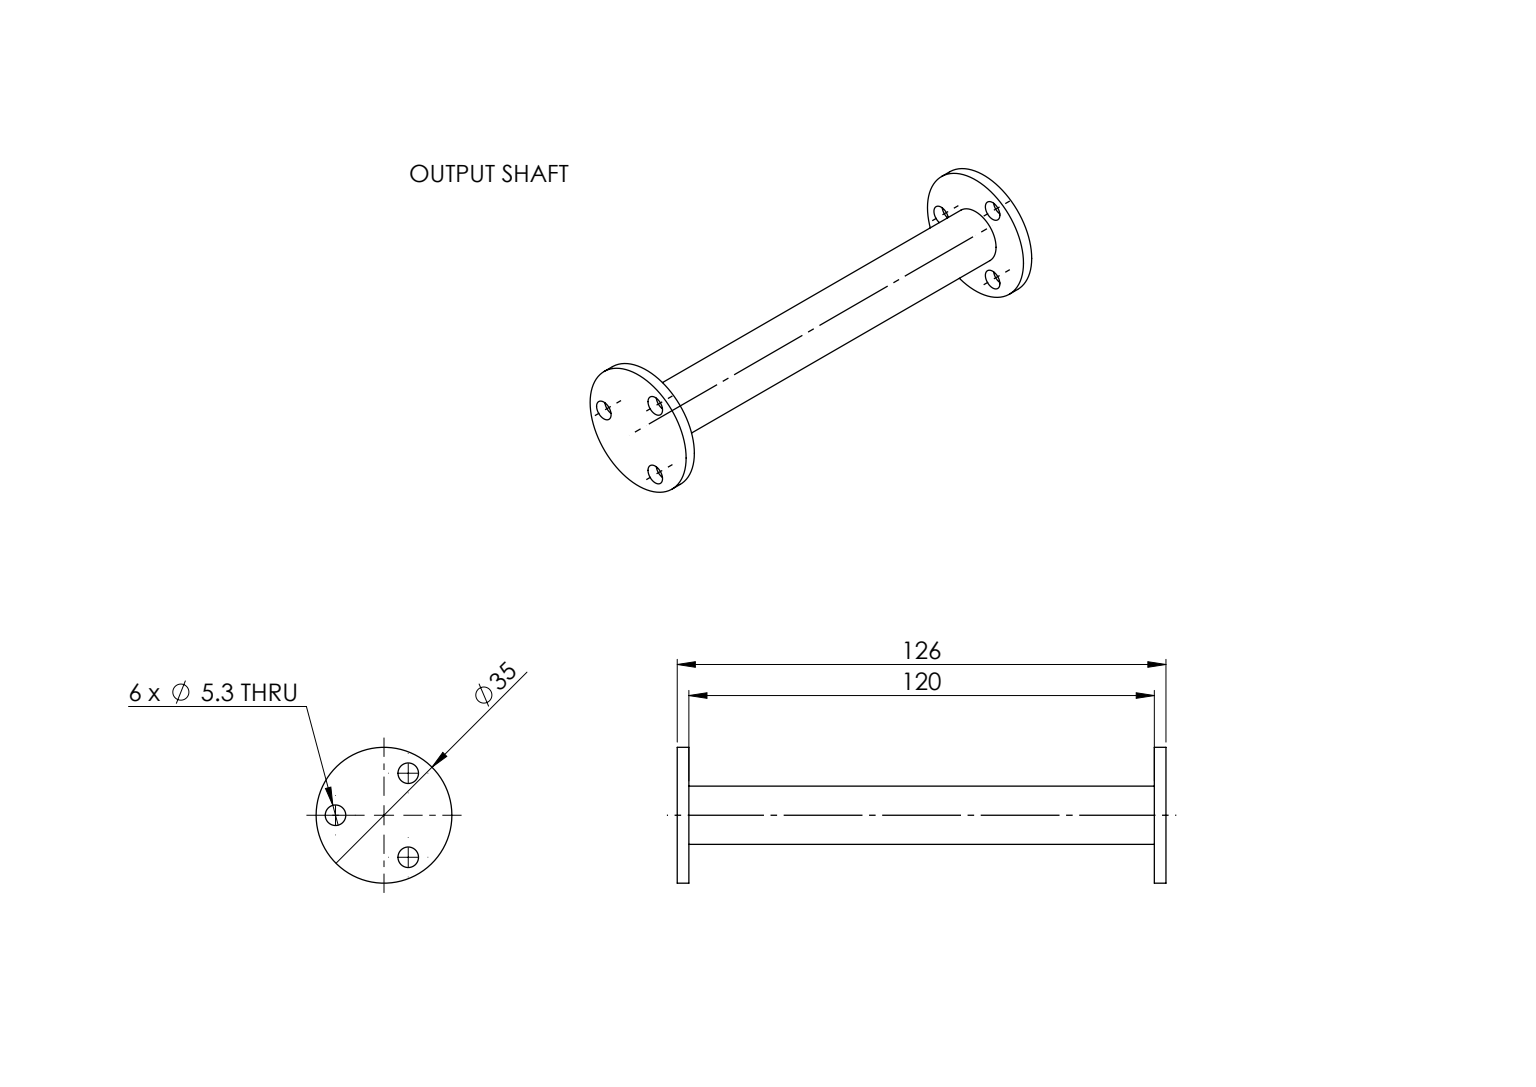
ISO-10303-21;
HEADER;
FILE_DESCRIPTION (('STEP AP214'),
    '1' );
FILE_NAME ('output shaft.step',
    '2026-10-03T12:29:21',
    ( '' ),
    ( '' ),
    'SwSTEP 2.0',
    'SolidWorks 2026',
    '' );
FILE_SCHEMA (( 'AUTOMOTIVE_DESIGN' ));
ENDSEC;

DATA;
#23=ORIENTED_EDGE ( 'NONE', *, *, #11876, .F. ) ;
#33=EDGE_CURVE ( 'NONE', #6658, #4014, #18101, .T. ) ;
#44=VERTEX_POINT ( 'NONE', #17992 ) ;
#49=EDGE_CURVE ( 'NONE', #12259, #9717, #8442, .T. ) ;
#118=ORIENTED_EDGE ( 'NONE', *, *, #9973, .F. ) ;
#146=ORIENTED_EDGE ( 'NONE', *, *, #3092, .T. ) ;
#154=EDGE_CURVE ( 'NONE', #4126, #11972, #18017, .T. ) ;
#178=AXIS2_PLACEMENT_3D ( 'NONE', #7554, #12660, #3003 ) ;
#185=DIRECTION ( 'NONE',  ( 1.000000000000000000, 0.000000000000000000, 0.000000000000000000 ) ) ;
#189=APPLICATION_CONTEXT ( 'automotive_design' ) ;
#208=VECTOR ( 'NONE', #12134, 1000.000000000000000 ) ;
#215=DIRECTION ( 'NONE',  ( 1.000000000000000000, 0.000000000000000000, 0.000000000000000000 ) ) ;
#279=FACE_BOUND ( 'NONE', #8489, .T. ) ;
#299=CARTESIAN_POINT ( 'NONE',  ( 0.000000000000000000, 0.000000000000000000, 46.00000000000000711 ) ) ;
#389=EDGE_LOOP ( 'NONE', ( #1248, #17136 ) ) ;
#393=DIRECTION ( 'NONE',  ( -0.000000000000000000, -0.000000000000000000, 1.000000000000000000 ) ) ;
#395=CYLINDRICAL_SURFACE ( 'NONE', #13106, 2.649999999999993694 ) ;
#396=CARTESIAN_POINT ( 'NONE',  ( 3.599999999999909051, -10.82531754730554496, 169.0000000000000000 ) ) ;
#416=PRESENTATION_STYLE_ASSIGNMENT (( #4000 ) ) ;
#432=ORIENTED_EDGE ( 'NONE', *, *, #14930, .F. ) ;
#509=ADVANCED_FACE ( 'NONE', ( #15936 ), #19629, .T. ) ;
#543=CARTESIAN_POINT ( 'NONE',  ( -15.15000000000000036, 0.000000000000000000, 166.0000000000000000 ) ) ;
#547=ORIENTED_EDGE ( 'NONE', *, *, #16992, .T. ) ;
#559=CARTESIAN_POINT ( 'NONE',  ( 7.500000000000000000, 9.184850993605147944E-16, 166.0000000000000000 ) ) ;
#615=DIRECTION ( 'NONE',  ( 0.000000000000000000, 0.000000000000000000, -1.000000000000000000 ) ) ;
#638=FACE_OUTER_BOUND ( 'NONE', #14639, .T. ) ;
#697=PRODUCT_DEFINITION_SHAPE ( 'NONE', 'NONE',  #15563 ) ;
#704=DIRECTION ( 'NONE',  ( 0.000000000000000000, 0.000000000000000000, 1.000000000000000000 ) ) ;
#709=CARTESIAN_POINT ( 'NONE',  ( 6.249999999999902300, -10.82531754730554496, 166.0000000000000000 ) ) ;
#762=ORIENTED_EDGE ( 'NONE', *, *, #14410, .F. ) ;
#773=FACE_OUTER_BOUND ( 'NONE', #9225, .T. ) ;
#774=CARTESIAN_POINT ( 'NONE',  ( 6.250000000000054179, 10.82531754730546147, 166.0000000000000000 ) ) ;
#798=VERTEX_POINT ( 'NONE', #3718 ) ;
#817=ORIENTED_EDGE ( 'NONE', *, *, #10804, .T. ) ;
#907=CARTESIAN_POINT ( 'NONE',  ( -15.14999999999999325, 3.245314017740474129E-16, 46.00000000000000711 ) ) ;
#967=DIRECTION ( 'NONE',  ( -0.000000000000000000, -0.000000000000000000, 1.000000000000000000 ) ) ;
#990=CARTESIAN_POINT ( 'NONE',  ( 17.50000000000000355, 2.143131898507868643E-15, 46.00000000000000711 ) ) ;
#994=DIRECTION ( 'NONE',  ( -0.000000000000000000, -0.000000000000000000, -1.000000000000000000 ) ) ;
#995=DIRECTION ( 'NONE',  ( 1.000000000000000000, 0.000000000000000000, -0.000000000000000000 ) ) ;
#1011=ADVANCED_FACE ( 'NONE', ( #9856 ), #8076, .T. ) ;
#1046=CARTESIAN_POINT ( 'NONE',  ( 6.249999999999902300, -10.82531754730554496, 46.00000000000000711 ) ) ;
#1071=DIRECTION ( 'NONE',  ( 1.000000000000000000, 0.000000000000000000, 0.000000000000000000 ) ) ;
#1183=FACE_OUTER_BOUND ( 'NONE', #6325, .T. ) ;
#1235=CARTESIAN_POINT ( 'NONE',  ( 6.250000000000054179, 10.82531754730546147, 46.00000000000000711 ) ) ;
#1241=AXIS2_PLACEMENT_3D ( 'NONE', #11873, #5718, #10613 ) ;
#1248=ORIENTED_EDGE ( 'NONE', *, *, #19286, .F. ) ;
#1272=CIRCLE ( 'NONE', #19871, 2.649999999999988365 ) ;
#1302=CARTESIAN_POINT ( 'NONE',  ( -12.50000000000000533, 0.000000000000000000, 166.0000000000000000 ) ) ;
#1303=VECTOR ( 'NONE', #20268, 1000.000000000000000 ) ;
#1342=ORIENTED_EDGE ( 'NONE', *, *, #18173, .T. ) ;
#1377=VERTEX_POINT ( 'NONE', #13674 ) ;
#1391=CIRCLE ( 'NONE', #8796, 2.649999999999987477 ) ;
#1396=DIRECTION ( 'NONE',  ( -0.000000000000000000, -0.000000000000000000, -1.000000000000000000 ) ) ;
#1436=CARTESIAN_POINT ( 'NONE',  ( 6.250000000000054179, 10.82531754730546147, 166.0000000000000000 ) ) ;
#1442=DIRECTION ( 'NONE',  ( -1.000000000000000000, 0.000000000000000000, 0.000000000000000000 ) ) ;
#1465=CARTESIAN_POINT ( 'NONE',  ( 0.000000000000000000, 0.000000000000000000, 46.00000000000000711 ) ) ;
#1537=CARTESIAN_POINT ( 'NONE',  ( -15.15000000000000036, 3.245314017740478073E-16, 46.00000000000000711 ) ) ;
#1566=DIRECTION ( 'NONE',  ( 0.000000000000000000, 0.000000000000000000, -1.000000000000000000 ) ) ;
#1584=EDGE_LOOP ( 'NONE', ( #432, #16666 ) ) ;
#1643=DIRECTION ( 'NONE',  ( -0.000000000000000000, -0.000000000000000000, 1.000000000000000000 ) ) ;
#1666=DIRECTION ( 'NONE',  ( 0.000000000000000000, 0.000000000000000000, 1.000000000000000000 ) ) ;
#1725=ORIENTED_EDGE ( 'NONE', *, *, #10894, .T. ) ;
#1730=EDGE_CURVE ( 'NONE', #8987, #10156, #13632, .T. ) ;
#1735=VECTOR ( 'NONE', #8612, 1000.000000000000000 ) ;
#1811=AXIS2_PLACEMENT_3D ( 'NONE', #3048, #20476, #8226 ) ;
#1851=EDGE_CURVE ( 'NONE', #4126, #9250, #2916, .T. ) ;
#1857=VERTEX_POINT ( 'NONE', #17557 ) ;
#1868=FACE_BOUND ( 'NONE', #1584, .T. ) ;
#1938=DIRECTION ( 'NONE',  ( 1.000000000000000000, 0.000000000000000000, 0.000000000000000000 ) ) ;
#2064=DIRECTION ( 'NONE',  ( -0.000000000000000000, -0.000000000000000000, -1.000000000000000000 ) ) ;
#2071=ORIENTED_EDGE ( 'NONE', *, *, #8027, .T. ) ;
#2128=DIRECTION ( 'NONE',  ( -0.000000000000000000, -0.000000000000000000, 1.000000000000000000 ) ) ;
#2198=ORIENTED_EDGE ( 'NONE', *, *, #20871, .T. ) ;
#2261=FACE_OUTER_BOUND ( 'NONE', #4125, .T. ) ;
#2269=DIRECTION ( 'NONE',  ( -0.000000000000000000, -0.000000000000000000, 1.000000000000000000 ) ) ;
#2396=VERTEX_POINT ( 'NONE', #14030 ) ;
#2454=ORIENTED_EDGE ( 'NONE', *, *, #15088, .T. ) ;
#2459=CIRCLE ( 'NONE', #14327, 2.649999999999993694 ) ;
#2464=COLOUR_RGB ( '', 0.40784314, 0.44705882, 0.49803922) ;
#2469=EDGE_LOOP ( 'NONE', ( #20521, #11520 ) ) ;
#2486=APPLICATION_CONTEXT ( 'automotive_design' ) ;
#2513=CYLINDRICAL_SURFACE ( 'NONE', #3801, 17.50000000000000355 ) ;
#2514=ORIENTED_EDGE ( 'NONE', *, *, #5799, .T. ) ;
#2545=CARTESIAN_POINT ( 'NONE',  ( 0.000000000000000000, 0.000000000000000000, 166.0000000000000000 ) ) ;
#2620=DIRECTION ( 'NONE',  ( 1.000000000000000000, 0.000000000000000000, 0.000000000000000000 ) ) ;
#2637=CARTESIAN_POINT ( 'NONE',  ( 3.600000000000060485, 10.82531754730546147, 46.00000000000000711 ) ) ;
#2682=DIRECTION ( 'NONE',  ( 0.000000000000000000, 0.000000000000000000, -1.000000000000000000 ) ) ;
#2703=ORIENTED_EDGE ( 'NONE', *, *, #3092, .F. ) ;
#2762=ADVANCED_FACE ( 'NONE', ( #1183 ), #20654, .F. ) ;
#2771=CARTESIAN_POINT ( 'NONE',  ( 6.249999999999902300, -10.82531754730554496, 169.0000000000000000 ) ) ;
#2822=CIRCLE ( 'NONE', #3156, 17.50000000000000355 ) ;
#2889=DIRECTION ( 'NONE',  ( 1.000000000000000000, 0.000000000000000000, 0.000000000000000000 ) ) ;
#2896=CARTESIAN_POINT ( 'NONE',  ( 3.599999999999909051, -10.82531754730554496, 166.0000000000000000 ) ) ;
#2916=LINE ( 'NONE', #12462, #17712 ) ;
#3003=DIRECTION ( 'NONE',  ( -1.000000000000000000, 0.000000000000000000, 0.000000000000000000 ) ) ;
#3016=CARTESIAN_POINT ( 'NONE',  ( 0.000000000000000000, 0.000000000000000000, 166.0000000000000000 ) ) ;
#3029=CARTESIAN_POINT ( 'NONE',  ( 8.900000000000046541, 10.82531754730546147, 46.00000000000000711 ) ) ;
#3042=FACE_BOUND ( 'NONE', #2469, .T. ) ;
#3048=CARTESIAN_POINT ( 'NONE',  ( 0.000000000000000000, 0.000000000000000000, 46.00000000000000711 ) ) ;
#3068=CARTESIAN_POINT ( 'NONE',  ( 0.000000000000000000, 0.000000000000000000, 46.00000000000000711 ) ) ;
#3075=SURFACE_STYLE_USAGE ( .BOTH. , #9333 ) ;
#3092=EDGE_CURVE ( 'NONE', #10942, #8932, #4499, .T. ) ;
#3107=VERTEX_POINT ( 'NONE', #18107 ) ;
#3121=CARTESIAN_POINT ( 'NONE',  ( 6.249999999999902300, -10.82531754730554496, 166.0000000000000000 ) ) ;
#3138=DIRECTION ( 'NONE',  ( 1.000000000000000000, 0.000000000000000000, 0.000000000000000000 ) ) ;
#3151=CYLINDRICAL_SURFACE ( 'NONE', #1811, 17.50000000000000355 ) ;
#3156=AXIS2_PLACEMENT_3D ( 'NONE', #18774, #7630, #1071 ) ;
#3177=ORIENTED_EDGE ( 'NONE', *, *, #19190, .T. ) ;
#3205=ORIENTED_EDGE ( 'NONE', *, *, #18428, .F. ) ;
#3260=ORIENTED_EDGE ( 'NONE', *, *, #18428, .T. ) ;
#3289=( GEOMETRIC_REPRESENTATION_CONTEXT ( 3 ) GLOBAL_UNCERTAINTY_ASSIGNED_CONTEXT ( ( #3895 ) ) GLOBAL_UNIT_ASSIGNED_CONTEXT ( ( #15899, #14325, #11028 ) ) REPRESENTATION_CONTEXT ( 'NONE', 'WORKASPACE' ) );
#3361=DIRECTION ( 'NONE',  ( 0.000000000000000000, 0.000000000000000000, 1.000000000000000000 ) ) ;
#3416=EDGE_LOOP ( 'NONE', ( #3205, #2703, #5913, #2514 ) ) ;
#3442=DIRECTION ( 'NONE',  ( -0.000000000000000000, -0.000000000000000000, 1.000000000000000000 ) ) ;
#3446=ORIENTED_EDGE ( 'NONE', *, *, #33, .T. ) ;
#3468=CARTESIAN_POINT ( 'NONE',  ( 0.000000000000000000, 0.000000000000000000, 166.0000000000000000 ) ) ;
#3469=ORIENTED_EDGE ( 'NONE', *, *, #5276, .F. ) ;
#3543=AXIS2_PLACEMENT_3D ( 'NONE', #6870, #20115, #11759 ) ;
#3576=ORIENTED_EDGE ( 'NONE', *, *, #16490, .F. ) ;
#3580=EDGE_LOOP ( 'NONE', ( #20126, #10307, #18630, #17660 ) ) ;
#3628=VERTEX_POINT ( 'NONE', #5103 ) ;
#3704=FACE_OUTER_BOUND ( 'NONE', #10097, .T. ) ;
#3718=CARTESIAN_POINT ( 'NONE',  ( 17.50000000000000355, 2.143131898507868643E-15, 46.00000000000000711 ) ) ;
#3739=ORIENTED_EDGE ( 'NONE', *, *, #13222, .T. ) ;
#3768=CARTESIAN_POINT ( 'NONE',  ( 6.250000000000054179, 10.82531754730546147, 169.0000000000000000 ) ) ;
#3769=ORIENTED_EDGE ( 'NONE', *, *, #18633, .T. ) ;
#3789=CYLINDRICAL_SURFACE ( 'NONE', #3543, 2.649999999999994582 ) ;
#3801=AXIS2_PLACEMENT_3D ( 'NONE', #14069, #6095, #2620 ) ;
#3837=AXIS2_PLACEMENT_3D ( 'NONE', #16417, #14627, #8066 ) ;
#3895=UNCERTAINTY_MEASURE_WITH_UNIT (LENGTH_MEASURE( 1.000000000000000082E-05 ), #15899, 'distance_accuracy_value', 'NONE');
#3896=( LENGTH_UNIT ( ) NAMED_UNIT ( * ) SI_UNIT ( .MILLI., .METRE. ) );
#3922=AXIS2_PLACEMENT_3D ( 'NONE', #17466, #5683, #10990 ) ;
#3972=VECTOR ( 'NONE', #20531, 1000.000000000000000 ) ;
#3984=DIRECTION ( 'NONE',  ( -1.000000000000000000, 0.000000000000000000, 0.000000000000000000 ) ) ;
#4000=SURFACE_STYLE_USAGE ( .BOTH. , #8460 ) ;
#4014=VERTEX_POINT ( 'NONE', #16776 ) ;
#4034=CIRCLE ( 'NONE', #13874, 2.649999999999993694 ) ;
#4044=EDGE_CURVE ( 'NONE', #10942, #3107, #12216, .T. ) ;
#4071=ADVANCED_FACE ( 'NONE', ( #773 ), #7223, .F. ) ;
#4112=FACE_BOUND ( 'NONE', #15261, .T. ) ;
#4118=CARTESIAN_POINT ( 'NONE',  ( 6.250000000000054179, 10.82531754730546147, 46.00000000000000711 ) ) ;
#4125=EDGE_LOOP ( 'NONE', ( #9380, #6892, #547, #14561 ) ) ;
#4126=VERTEX_POINT ( 'NONE', #16667 ) ;
#4142=CARTESIAN_POINT ( 'NONE',  ( -7.500000000000000000, 0.000000000000000000, 166.0000000000000000 ) ) ;
#4175=VERTEX_POINT ( 'NONE', #20587 ) ;
#4182=ORIENTED_EDGE ( 'NONE', *, *, #1730, .T. ) ;
#4262=ADVANCED_FACE ( 'NONE', ( #14347, #12536, #10943, #17421 ), #14032, .F. ) ;
#4281=AXIS2_PLACEMENT_3D ( 'NONE', #2771, #7752, #12315 ) ;
#4391=DIRECTION ( 'NONE',  ( 1.000000000000000000, 0.000000000000000000, 0.000000000000000000 ) ) ;
#4404=EDGE_CURVE ( 'NONE', #7823, #16612, #10879, .T. ) ;
#4413=CARTESIAN_POINT ( 'NONE',  ( -12.50000000000000533, 0.000000000000000000, 43.00000000000000000 ) ) ;
#4457=DIRECTION ( 'NONE',  ( -1.000000000000000000, 0.000000000000000000, 0.000000000000000000 ) ) ;
#4493=DIRECTION ( 'NONE',  ( 0.000000000000000000, 0.000000000000000000, 1.000000000000000000 ) ) ;
#4499=CIRCLE ( 'NONE', #11590, 7.500000000000000000 ) ;
#4539=EDGE_CURVE ( 'NONE', #13894, #12404, #10608, .T. ) ;
#4547=CARTESIAN_POINT ( 'NONE',  ( 3.600000000000060485, 10.82531754730546147, 166.0000000000000000 ) ) ;
#4551=VERTEX_POINT ( 'NONE', #15482 ) ;
#4558=ORIENTED_EDGE ( 'NONE', *, *, #10782, .F. ) ;
#4575=CARTESIAN_POINT ( 'NONE',  ( -12.50000000000000533, 0.000000000000000000, 46.00000000000000711 ) ) ;
#4577=ADVANCED_FACE ( 'NONE', ( #3704 ), #16640, .F. ) ;
#4591=ORIENTED_EDGE ( 'NONE', *, *, #13216, .T. ) ;
#4595=DIRECTION ( 'NONE',  ( -0.000000000000000000, -0.000000000000000000, 1.000000000000000000 ) ) ;
#4609=DIRECTION ( 'NONE',  ( -0.000000000000000000, -0.000000000000000000, -1.000000000000000000 ) ) ;
#4684=CARTESIAN_POINT ( 'NONE',  ( 0.000000000000000000, 0.000000000000000000, 166.0000000000000000 ) ) ;
#4797=CARTESIAN_POINT ( 'NONE',  ( -12.50000000000000533, 0.000000000000000000, 46.00000000000000711 ) ) ;
#4806=ORIENTED_EDGE ( 'NONE', *, *, #5276, .T. ) ;
#4864=CIRCLE ( 'NONE', #9275, 17.50000000000000355 ) ;
#4869=ORIENTED_EDGE ( 'NONE', *, *, #14144, .T. ) ;
#4889=VECTOR ( 'NONE', #18790, 1000.000000000000000 ) ;
#4890=ORIENTED_EDGE ( 'NONE', *, *, #4404, .T. ) ;
#4919=ORIENTED_EDGE ( 'NONE', *, *, #6891, .F. ) ;
#4936=DIRECTION ( 'NONE',  ( 1.000000000000000000, 0.000000000000000000, 0.000000000000000000 ) ) ;
#4939=CIRCLE ( 'NONE', #1241, 7.500000000000000000 ) ;
#4946=CIRCLE ( 'NONE', #7655, 2.649999999999994582 ) ;
#4981=CIRCLE ( 'NONE', #8693, 2.649999999999992806 ) ;
#5015=DIRECTION ( 'NONE',  ( -0.000000000000000000, -0.000000000000000000, -1.000000000000000000 ) ) ;
#5022=ORIENTED_EDGE ( 'NONE', *, *, #12228, .T. ) ;
#5091=ORIENTED_EDGE ( 'NONE', *, *, #19830, .T. ) ;
#5103=CARTESIAN_POINT ( 'NONE',  ( -17.50000000000000355, 0.000000000000000000, 46.00000000000000711 ) ) ;
#5126=EDGE_CURVE ( 'NONE', #1377, #20902, #5791, .T. ) ;
#5153=EDGE_LOOP ( 'NONE', ( #17444, #7861 ) ) ;
#5161=CYLINDRICAL_SURFACE ( 'NONE', #14138, 2.649999999999992806 ) ;
#5219=ORIENTED_EDGE ( 'NONE', *, *, #1851, .F. ) ;
#5260=SHAPE_DEFINITION_REPRESENTATION ( #697, #7225 ) ;
#5276=EDGE_CURVE ( 'NONE', #4175, #7756, #6527, .T. ) ;
#5278=ORIENTED_EDGE ( 'NONE', *, *, #11450, .T. ) ;
#5287=CARTESIAN_POINT ( 'NONE',  ( 6.249999999999902300, -10.82531754730554496, 46.00000000000000711 ) ) ;
#5299=ORIENTED_EDGE ( 'NONE', *, *, #6455, .T. ) ;
#5471=VERTEX_POINT ( 'NONE', #14141 ) ;
#5485=DIRECTION ( 'NONE',  ( -0.000000000000000000, -0.000000000000000000, 1.000000000000000000 ) ) ;
#5490=VECTOR ( 'NONE', #16397, 1000.000000000000000 ) ;
#5516=DIRECTION ( 'NONE',  ( -0.000000000000000000, -0.000000000000000000, 1.000000000000000000 ) ) ;
#5545=CIRCLE ( 'NONE', #15717, 2.649999999999987477 ) ;
#5560=CARTESIAN_POINT ( 'NONE',  ( 6.250000000000054179, 10.82531754730546147, 169.0000000000000000 ) ) ;
#5575=FACE_OUTER_BOUND ( 'NONE', #11083, .T. ) ;
#5585=ADVANCED_FACE ( 'NONE', ( #14458, #9256, #15719, #6168 ), #14037, .F. ) ;
#5593=FILL_AREA_STYLE ('',( #7293 ) ) ;
#5655=AXIS2_PLACEMENT_3D ( 'NONE', #4118, #967, #9216 ) ;
#5683=DIRECTION ( 'NONE',  ( 0.000000000000000000, 0.000000000000000000, 1.000000000000000000 ) ) ;
#5699=DIRECTION ( 'NONE',  ( 1.000000000000000000, 0.000000000000000000, 0.000000000000000000 ) ) ;
#5718=DIRECTION ( 'NONE',  ( 0.000000000000000000, 0.000000000000000000, 1.000000000000000000 ) ) ;
#5748=DIRECTION ( 'NONE',  ( 1.000000000000000000, 0.000000000000000000, 0.000000000000000000 ) ) ;
#5767=VECTOR ( 'NONE', #18249, 1000.000000000000000 ) ;
#5791=LINE ( 'NONE', #2637, #12935 ) ;
#5799=EDGE_CURVE ( 'NONE', #3107, #6625, #4939, .T. ) ;
#5806=ORIENTED_EDGE ( 'NONE', *, *, #10782, .T. ) ;
#5846=CARTESIAN_POINT ( 'NONE',  ( -15.14999999999999325, 0.000000000000000000, 166.0000000000000000 ) ) ;
#5863=CARTESIAN_POINT ( 'NONE',  ( -12.50000000000000533, 0.000000000000000000, 46.00000000000000711 ) ) ;
#5913=ORIENTED_EDGE ( 'NONE', *, *, #4044, .T. ) ;
#5934=CARTESIAN_POINT ( 'NONE',  ( 6.249999999999902300, -10.82531754730554496, 46.00000000000000711 ) ) ;
#5950=VERTEX_POINT ( 'NONE', #12191 ) ;
#5972=AXIS2_PLACEMENT_3D ( 'NONE', #299, #7944, #9935 ) ;
#6038=ORIENTED_EDGE ( 'NONE', *, *, #14554, .T. ) ;
#6095=DIRECTION ( 'NONE',  ( -0.000000000000000000, -0.000000000000000000, 1.000000000000000000 ) ) ;
#6123=DIRECTION ( 'NONE',  ( -0.000000000000000000, -0.000000000000000000, 1.000000000000000000 ) ) ;
#6140=DIRECTION ( 'NONE',  ( -0.000000000000000000, -0.000000000000000000, -1.000000000000000000 ) ) ;
#6168=FACE_OUTER_BOUND ( 'NONE', #19328, .T. ) ;
#6183=CARTESIAN_POINT ( 'NONE',  ( 0.000000000000000000, 0.000000000000000000, 46.00000000000000711 ) ) ;
#6232=CARTESIAN_POINT ( 'NONE',  ( 0.000000000000000000, 0.000000000000000000, 169.0000000000000000 ) ) ;
#6271=ORIENTED_EDGE ( 'NONE', *, *, #8978, .F. ) ;
#6296=DIRECTION ( 'NONE',  ( -1.000000000000000000, 0.000000000000000000, 0.000000000000000000 ) ) ;
#6319=DIRECTION ( 'NONE',  ( 1.000000000000000000, 0.000000000000000000, 0.000000000000000000 ) ) ;
#6325=EDGE_LOOP ( 'NONE', ( #13791, #15376, #7809, #5299 ) ) ;
#6331=CARTESIAN_POINT ( 'NONE',  ( 3.599999999999909051, -10.82531754730554496, 43.00000000000000000 ) ) ;
#6390=CARTESIAN_POINT ( 'NONE',  ( -17.50000000000000355, 2.143131898507868643E-15, 169.0000000000000000 ) ) ;
#6393=CARTESIAN_POINT ( 'NONE',  ( 8.899999999999895550, -10.82531754730554496, 166.0000000000000000 ) ) ;
#6410=DIRECTION ( 'NONE',  ( 1.000000000000000000, 0.000000000000000000, 0.000000000000000000 ) ) ;
#6414=FACE_OUTER_BOUND ( 'NONE', #5153, .T. ) ;
#6455=EDGE_CURVE ( 'NONE', #9717, #4014, #1272, .T. ) ;
#6517=DIRECTION ( 'NONE',  ( -1.000000000000000000, 0.000000000000000000, 0.000000000000000000 ) ) ;
#6527=LINE ( 'NONE', #13012, #9683 ) ;
#6547=CIRCLE ( 'NONE', #20777, 2.649999999999994582 ) ;
#6625=VERTEX_POINT ( 'NONE', #18092 ) ;
#6627=CIRCLE ( 'NONE', #15098, 17.50000000000000355 ) ;
#6630=FACE_OUTER_BOUND ( 'NONE', #20266, .T. ) ;
#6658=VERTEX_POINT ( 'NONE', #6331 ) ;
#6705=DIRECTION ( 'NONE',  ( -1.000000000000000000, 0.000000000000000000, 0.000000000000000000 ) ) ;
#6759=EDGE_LOOP ( 'NONE', ( #18853, #4558 ) ) ;
#6812=CARTESIAN_POINT ( 'NONE',  ( 8.900000000000041211, 10.82531754730546147, 166.0000000000000000 ) ) ;
#6849=DIRECTION ( 'NONE',  ( -0.000000000000000000, -0.000000000000000000, -1.000000000000000000 ) ) ;
#6870=CARTESIAN_POINT ( 'NONE',  ( -12.50000000000000533, 0.000000000000000000, 166.0000000000000000 ) ) ;
#6891=EDGE_CURVE ( 'NONE', #6658, #12259, #16502, .T. ) ;
#6892=ORIENTED_EDGE ( 'NONE', *, *, #1851, .T. ) ;
#6962=ORIENTED_EDGE ( 'NONE', *, *, #12398, .T. ) ;
#6971=DIRECTION ( 'NONE',  ( 0.000000000000000000, 0.000000000000000000, -1.000000000000000000 ) ) ;
#7114=EDGE_LOOP ( 'NONE', ( #3469, #14583, #16857, #5022 ) ) ;
#7223=CYLINDRICAL_SURFACE ( 'NONE', #18996, 2.649999999999993694 ) ;
#7225=SHAPE_REPRESENTATION ( 'output shaft', ( #12461 ), #8672 ) ;
#7232=AXIS2_PLACEMENT_3D ( 'NONE', #1235, #7888, #4391 ) ;
#7261=ORIENTED_EDGE ( 'NONE', *, *, #11450, .F. ) ;
#7290=EDGE_CURVE ( 'NONE', #13088, #5950, #7342, .T. ) ;
#7293=FILL_AREA_STYLE_COLOUR ( '', #2464 ) ;
#7342=LINE ( 'NONE', #2896, #1303 ) ;
#7358=CARTESIAN_POINT ( 'NONE',  ( 0.000000000000000000, 0.000000000000000000, 46.00000000000000711 ) ) ;
#7373=ORIENTED_EDGE ( 'NONE', *, *, #10229, .T. ) ;
#7420=CYLINDRICAL_SURFACE ( 'NONE', #19400, 2.649999999999994582 ) ;
#7438=CARTESIAN_POINT ( 'NONE',  ( -7.500000000000000000, 0.000000000000000000, 166.0000000000000000 ) ) ;
#7490=ORIENTED_EDGE ( 'NONE', *, *, #15962, .T. ) ;
#7522=DIRECTION ( 'NONE',  ( -1.000000000000000000, 0.000000000000000000, 0.000000000000000000 ) ) ;
#7554=CARTESIAN_POINT ( 'NONE',  ( -12.50000000000000533, 0.000000000000000000, 166.0000000000000000 ) ) ;
#7563=LINE ( 'NONE', #1537, #12722 ) ;
#7567=DIRECTION ( 'NONE',  ( 1.000000000000000000, 0.000000000000000000, 0.000000000000000000 ) ) ;
#7630=DIRECTION ( 'NONE',  ( 0.000000000000000000, 0.000000000000000000, 1.000000000000000000 ) ) ;
#7635=PRESENTATION_STYLE_ASSIGNMENT (( #3075 ) ) ;
#7655=AXIS2_PLACEMENT_3D ( 'NONE', #4413, #9296, #6319 ) ;
#7714=CARTESIAN_POINT ( 'NONE',  ( -9.850000000000012079, 0.000000000000000000, 43.00000000000000000 ) ) ;
#7752=DIRECTION ( 'NONE',  ( 0.000000000000000000, 0.000000000000000000, -1.000000000000000000 ) ) ;
#7756=VERTEX_POINT ( 'NONE', #15042 ) ;
#7767=CARTESIAN_POINT ( 'NONE',  ( 0.000000000000000000, 0.000000000000000000, 43.00000000000000000 ) ) ;
#7808=AXIS2_PLACEMENT_3D ( 'NONE', #19114, #2682, #2889 ) ;
#7809=ORIENTED_EDGE ( 'NONE', *, *, #49, .T. ) ;
#7823=VERTEX_POINT ( 'NONE', #17476 ) ;
#7836=EDGE_LOOP ( 'NONE', ( #11884, #20659, #5278, #16232 ) ) ;
#7844=SURFACE_STYLE_FILL_AREA ( #16118 ) ;
#7852=DIRECTION ( 'NONE',  ( -1.000000000000000000, 0.000000000000000000, 0.000000000000000000 ) ) ;
#7861=ORIENTED_EDGE ( 'NONE', *, *, #14807, .F. ) ;
#7872=CLOSED_SHELL ( 'NONE', ( #15585, #13504, #4071, #16328, #15702, #13043, #4577, #1011, #14306, #14016, #20326, #5585, #8284, #2762, #12749, #9733, #509, #19068, #4262, #20002, #12008, #10242 ) ) ;
#7888=DIRECTION ( 'NONE',  ( -0.000000000000000000, -0.000000000000000000, 1.000000000000000000 ) ) ;
#7919=EDGE_LOOP ( 'NONE', ( #3739, #12021 ) ) ;
#7944=DIRECTION ( 'NONE',  ( 0.000000000000000000, 0.000000000000000000, 1.000000000000000000 ) ) ;
#7988=AXIS2_PLACEMENT_3D ( 'NONE', #7767, #18910, #12862 ) ;
#8014=VERTEX_POINT ( 'NONE', #18714 ) ;
#8027=EDGE_CURVE ( 'NONE', #8014, #5950, #18346, .T. ) ;
#8066=DIRECTION ( 'NONE',  ( 1.000000000000000000, 0.000000000000000000, 0.000000000000000000 ) ) ;
#8076=CYLINDRICAL_SURFACE ( 'NONE', #20008, 7.500000000000000000 ) ;
#8125=ORIENTED_EDGE ( 'NONE', *, *, #11555, .T. ) ;
#8188=DIRECTION ( 'NONE',  ( -0.000000000000000000, -0.000000000000000000, -1.000000000000000000 ) ) ;
#8193=DIRECTION ( 'NONE',  ( 1.000000000000000000, 0.000000000000000000, 0.000000000000000000 ) ) ;
#8226=DIRECTION ( 'NONE',  ( -1.000000000000000000, 0.000000000000000000, 0.000000000000000000 ) ) ;
#8239=CARTESIAN_POINT ( 'NONE',  ( 3.599999999999909051, -10.82531754730554496, 46.00000000000000711 ) ) ;
#8241=EDGE_LOOP ( 'NONE', ( #9081, #13985, #11177, #11832 ) ) ;
#8265=DIRECTION ( 'NONE',  ( 0.000000000000000000, 0.000000000000000000, 1.000000000000000000 ) ) ;
#8278=ORIENTED_EDGE ( 'NONE', *, *, #14144, .F. ) ;
#8284=ADVANCED_FACE ( 'NONE', ( #8669 ), #11756, .T. ) ;
#8394=LINE ( 'NONE', #6393, #15019 ) ;
#8442=LINE ( 'NONE', #16511, #13616 ) ;
#8444=EDGE_LOOP ( 'NONE', ( #17812, #23, #11731, #4869 ) ) ;
#8460=SURFACE_SIDE_STYLE ('',( #8881 ) ) ;
#8489=EDGE_LOOP ( 'NONE', ( #17044, #762 ) ) ;
#8526=ORIENTED_EDGE ( 'NONE', *, *, #17670, .T. ) ;
#8547=( GEOMETRIC_REPRESENTATION_CONTEXT ( 3 ) GLOBAL_UNCERTAINTY_ASSIGNED_CONTEXT ( ( #15356 ) ) GLOBAL_UNIT_ASSIGNED_CONTEXT ( ( #3896, #10482, #16938 ) ) REPRESENTATION_CONTEXT ( 'NONE', 'WORKASPACE' ) );
#8576=AXIS2_PLACEMENT_3D ( 'NONE', #6232, #6123, #9207 ) ;
#8594=VECTOR ( 'NONE', #4595, 1000.000000000000000 ) ;
#8612=DIRECTION ( 'NONE',  ( -0.000000000000000000, -0.000000000000000000, -1.000000000000000000 ) ) ;
#8669=FACE_OUTER_BOUND ( 'NONE', #3416, .T. ) ;
#8672=( GEOMETRIC_REPRESENTATION_CONTEXT ( 3 ) GLOBAL_UNCERTAINTY_ASSIGNED_CONTEXT ( ( #8773 ) ) GLOBAL_UNIT_ASSIGNED_CONTEXT ( ( #10725, #18660, #12938 ) ) REPRESENTATION_CONTEXT ( 'NONE', 'WORKASPACE' ) );
#8693=AXIS2_PLACEMENT_3D ( 'NONE', #11655, #8265, #215 ) ;
#8734=CARTESIAN_POINT ( 'NONE',  ( -17.50000000000000355, 0.000000000000000000, 43.00000000000000000 ) ) ;
#8760=DIRECTION ( 'NONE',  ( 1.000000000000000000, 0.000000000000000000, 0.000000000000000000 ) ) ;
#8773=UNCERTAINTY_MEASURE_WITH_UNIT (LENGTH_MEASURE( 1.000000000000000082E-05 ), #10725, 'distance_accuracy_value', 'NONE');
#8774=FACE_OUTER_BOUND ( 'NONE', #7114, .T. ) ;
#8796=AXIS2_PLACEMENT_3D ( 'NONE', #19127, #8188, #9471 ) ;
#8866=AXIS2_PLACEMENT_3D ( 'NONE', #15144, #15043, #11851 ) ;
#8871=AXIS2_PLACEMENT_3D ( 'NONE', #3768, #615, #3984 ) ;
#8881=SURFACE_STYLE_FILL_AREA ( #5593 ) ;
#8932=VERTEX_POINT ( 'NONE', #12040 ) ;
#8962=EDGE_CURVE ( 'NONE', #11972, #4126, #2459, .T. ) ;
#8978=EDGE_CURVE ( 'NONE', #13237, #4551, #20712, .T. ) ;
#8987=VERTEX_POINT ( 'NONE', #9395 ) ;
#9014=DIRECTION ( 'NONE',  ( -0.000000000000000000, -0.000000000000000000, -1.000000000000000000 ) ) ;
#9033=DIRECTION ( 'NONE',  ( 1.000000000000000000, 0.000000000000000000, 0.000000000000000000 ) ) ;
#9081=ORIENTED_EDGE ( 'NONE', *, *, #18173, .F. ) ;
#9132=DIRECTION ( 'NONE',  ( -0.000000000000000000, -0.000000000000000000, 1.000000000000000000 ) ) ;
#9207=DIRECTION ( 'NONE',  ( 1.000000000000000000, 0.000000000000000000, 0.000000000000000000 ) ) ;
#9216=DIRECTION ( 'NONE',  ( 1.000000000000000000, 0.000000000000000000, 0.000000000000000000 ) ) ;
#9225=EDGE_LOOP ( 'NONE', ( #10634, #1342, #2071, #10842 ) ) ;
#9239=DIRECTION ( 'NONE',  ( -0.000000000000000000, -0.000000000000000000, 1.000000000000000000 ) ) ;
#9250=VERTEX_POINT ( 'NONE', #6812 ) ;
#9256=FACE_BOUND ( 'NONE', #7919, .T. ) ;
#9275=AXIS2_PLACEMENT_3D ( 'NONE', #18151, #5516, #10510 ) ;
#9278=CARTESIAN_POINT ( 'NONE',  ( 0.000000000000000000, 0.000000000000000000, 166.0000000000000000 ) ) ;
#9290=EDGE_LOOP ( 'NONE', ( #10881, #817 ) ) ;
#9296=DIRECTION ( 'NONE',  ( 0.000000000000000000, 0.000000000000000000, 1.000000000000000000 ) ) ;
#9319=CIRCLE ( 'NONE', #178, 2.649999999999987477 ) ;
#9333=SURFACE_SIDE_STYLE ('',( #7844 ) ) ;
#9373=MECHANICAL_DESIGN_GEOMETRIC_PRESENTATION_REPRESENTATION('',(#16807),#3289);
#9380=ORIENTED_EDGE ( 'NONE', *, *, #154, .F. ) ;
#9395=CARTESIAN_POINT ( 'NONE',  ( 17.50000000000000355, 0.000000000000000000, 166.0000000000000000 ) ) ;
#9411=AXIS2_PLACEMENT_3D ( 'NONE', #774, #18365, #10525 ) ;
#9429=ORIENTED_EDGE ( 'NONE', *, *, #10672, .F. ) ;
#9443=DIRECTION ( 'NONE',  ( -0.000000000000000000, -0.000000000000000000, -1.000000000000000000 ) ) ;
#9446=CARTESIAN_POINT ( 'NONE',  ( -12.50000000000000533, 0.000000000000000000, 169.0000000000000000 ) ) ;
#9471=DIRECTION ( 'NONE',  ( -1.000000000000000000, 0.000000000000000000, 0.000000000000000000 ) ) ;
#9595=DIRECTION ( 'NONE',  ( -0.000000000000000000, -0.000000000000000000, 1.000000000000000000 ) ) ;
#9609=LINE ( 'NONE', #12900, #11724 ) ;
#9614=FACE_OUTER_BOUND ( 'NONE', #19299, .T. ) ;
#9654=FILL_AREA_STYLE_COLOUR ( '', #18864 ) ;
#9683=VECTOR ( 'NONE', #12814, 1000.000000000000000 ) ;
#9717=VERTEX_POINT ( 'NONE', #11675 ) ;
#9733=ADVANCED_FACE ( 'NONE', ( #13172 ), #16148, .F. ) ;
#9738=ORIENTED_EDGE ( 'NONE', *, *, #154, .T. ) ;
#9756=FACE_OUTER_BOUND ( 'NONE', #3580, .T. ) ;
#9856=FACE_OUTER_BOUND ( 'NONE', #17380, .T. ) ;
#9906=ORIENTED_EDGE ( 'NONE', *, *, #19332, .F. ) ;
#9935=DIRECTION ( 'NONE',  ( 1.000000000000000000, 0.000000000000000000, 0.000000000000000000 ) ) ;
#9973=EDGE_CURVE ( 'NONE', #2396, #9250, #13303, .T. ) ;
#10036=PRODUCT_CONTEXT ( 'NONE', #2486, 'mechanical' ) ;
#10097=EDGE_LOOP ( 'NONE', ( #4919, #3446, #7373, #14134 ) ) ;
#10152=DIRECTION ( 'NONE',  ( 1.000000000000000000, 0.000000000000000000, 0.000000000000000000 ) ) ;
#10156=VERTEX_POINT ( 'NONE', #13151 ) ;
#10174=ORIENTED_EDGE ( 'NONE', *, *, #14410, .T. ) ;
#10194=MANIFOLD_SOLID_BREP ( 'Mirror1', #7872 ) ;
#10229=EDGE_CURVE ( 'NONE', #4014, #9717, #16963, .T. ) ;
#10242=ADVANCED_FACE ( 'NONE', ( #8774 ), #3789, .F. ) ;
#10286=ORIENTED_EDGE ( 'NONE', *, *, #15884, .T. ) ;
#10291=CARTESIAN_POINT ( 'NONE',  ( -15.15000000000000036, 0.000000000000000000, 169.0000000000000000 ) ) ;
#10307=ORIENTED_EDGE ( 'NONE', *, *, #10672, .T. ) ;
#10323=PRODUCT_DEFINITION_FORMATION_WITH_SPECIFIED_SOURCE ( 'ANY', '', #13215, .NOT_KNOWN. ) ;
#10349=ORIENTED_EDGE ( 'NONE', *, *, #8978, .T. ) ;
#10409=AXIS2_PLACEMENT_3D ( 'NONE', #13001, #2064, #6517 ) ;
#10458=ORIENTED_EDGE ( 'NONE', *, *, #16992, .F. ) ;
#10460=EDGE_LOOP ( 'NONE', ( #13477, #4806, #5806, #11847 ) ) ;
#10482=( NAMED_UNIT ( * ) PLANE_ANGLE_UNIT ( ) SI_UNIT ( $, .RADIAN. ) );
#10510=DIRECTION ( 'NONE',  ( 1.000000000000000000, 0.000000000000000000, 0.000000000000000000 ) ) ;
#10525=DIRECTION ( 'NONE',  ( -1.000000000000000000, 0.000000000000000000, 0.000000000000000000 ) ) ;
#10581=EDGE_LOOP ( 'NONE', ( #3177, #7490 ) ) ;
#10598=FACE_BOUND ( 'NONE', #14067, .T. ) ;
#10605=VERTEX_POINT ( 'NONE', #6390 ) ;
#10608=LINE ( 'NONE', #543, #19334 ) ;
#10610=ORIENTED_EDGE ( 'NONE', *, *, #5126, .T. ) ;
#10613=DIRECTION ( 'NONE',  ( 1.000000000000000000, 0.000000000000000000, 0.000000000000000000 ) ) ;
#10634=ORIENTED_EDGE ( 'NONE', *, *, #15884, .F. ) ;
#10671=DIRECTION ( 'NONE',  ( 1.000000000000000000, 0.000000000000000000, 0.000000000000000000 ) ) ;
#10672=EDGE_CURVE ( 'NONE', #11249, #11867, #7563, .T. ) ;
#10690=AXIS2_PLACEMENT_3D ( 'NONE', #20355, #9239, #9033 ) ;
#10718=CYLINDRICAL_SURFACE ( 'NONE', #14460, 17.50000000000000355 ) ;
#10720=ORIENTED_EDGE ( 'NONE', *, *, #8962, .F. ) ;
#10725=( LENGTH_UNIT ( ) NAMED_UNIT ( * ) SI_UNIT ( .MILLI., .METRE. ) );
#10773=ORIENTED_EDGE ( 'NONE', *, *, #6891, .T. ) ;
#10782=EDGE_CURVE ( 'NONE', #7756, #12404, #9319, .T. ) ;
#10790=LINE ( 'NONE', #20304, #3972 ) ;
#10792=ORIENTED_EDGE ( 'NONE', *, *, #16490, .T. ) ;
#10804=EDGE_CURVE ( 'NONE', #4175, #13894, #13724, .T. ) ;
#10842=ORIENTED_EDGE ( 'NONE', *, *, #7290, .F. ) ;
#10850=DIRECTION ( 'NONE',  ( -0.000000000000000000, -0.000000000000000000, 1.000000000000000000 ) ) ;
#10879=CIRCLE ( 'NONE', #12225, 17.50000000000000355 ) ;
#10881=ORIENTED_EDGE ( 'NONE', *, *, #17373, .T. ) ;
#10894=EDGE_CURVE ( 'NONE', #4551, #20902, #19806, .T. ) ;
#10930=AXIS2_PLACEMENT_3D ( 'NONE', #13098, #1666, #6410 ) ;
#10942=VERTEX_POINT ( 'NONE', #4142 ) ;
#10943=FACE_BOUND ( 'NONE', #18792, .T. ) ;
#10951=LINE ( 'NONE', #18913, #8594 ) ;
#10970=DIRECTION ( 'NONE',  ( 1.000000000000000000, 0.000000000000000000, 0.000000000000000000 ) ) ;
#10990=DIRECTION ( 'NONE',  ( 1.000000000000000000, 0.000000000000000000, 0.000000000000000000 ) ) ;
#11010=AXIS2_PLACEMENT_3D ( 'NONE', #12442, #20687, #14355 ) ;
#11028=( NAMED_UNIT ( * ) SI_UNIT ( $, .STERADIAN. ) SOLID_ANGLE_UNIT ( ) );
#11083=EDGE_LOOP ( 'NONE', ( #19083, #10610, #12108, #6271 ) ) ;
#11177=ORIENTED_EDGE ( 'NONE', *, *, #7290, .T. ) ;
#11209=ADVANCED_BREP_SHAPE_REPRESENTATION ( '', ( #10194, #12461 ), #8672 ) ;
#11249=VERTEX_POINT ( 'NONE', #13469 ) ;
#11363=CARTESIAN_POINT ( 'NONE',  ( 0.000000000000000000, 0.000000000000000000, 43.00000000000000000 ) ) ;
#11380=CIRCLE ( 'NONE', #10409, 2.649999999999988365 ) ;
#11450=EDGE_CURVE ( 'NONE', #8987, #44, #9609, .T. ) ;
#11452=CYLINDRICAL_SURFACE ( 'NONE', #3837, 2.649999999999994582 ) ;
#11520=ORIENTED_EDGE ( 'NONE', *, *, #11968, .F. ) ;
#11555=EDGE_CURVE ( 'NONE', #13182, #11249, #4946, .T. ) ;
#11590=AXIS2_PLACEMENT_3D ( 'NONE', #3468, #18214, #10152 ) ;
#11644=CIRCLE ( 'NONE', #18412, 2.649999999999987477 ) ;
#11655=CARTESIAN_POINT ( 'NONE',  ( 6.250000000000054179, 10.82531754730546147, 43.00000000000000000 ) ) ;
#11675=CARTESIAN_POINT ( 'NONE',  ( 8.899999999999890221, -10.82531754730554496, 46.00000000000000711 ) ) ;
#11689=DIRECTION ( 'NONE',  ( -0.000000000000000000, -0.000000000000000000, -1.000000000000000000 ) ) ;
#11724=VECTOR ( 'NONE', #17352, 1000.000000000000000 ) ;
#11731=ORIENTED_EDGE ( 'NONE', *, *, #19332, .T. ) ;
#11753=AXIS2_PLACEMENT_3D ( 'NONE', #1465, #13316, #995 ) ;
#11756=CYLINDRICAL_SURFACE ( 'NONE', #8866, 7.500000000000000000 ) ;
#11759=DIRECTION ( 'NONE',  ( -1.000000000000000000, 0.000000000000000000, 0.000000000000000000 ) ) ;
#11832=ORIENTED_EDGE ( 'NONE', *, *, #19286, .T. ) ;
#11838=EDGE_LOOP ( 'NONE', ( #9429, #13125, #2454, #14094 ) ) ;
#11847=ORIENTED_EDGE ( 'NONE', *, *, #4539, .F. ) ;
#11851=DIRECTION ( 'NONE',  ( -1.000000000000000000, 0.000000000000000000, 0.000000000000000000 ) ) ;
#11867=VERTEX_POINT ( 'NONE', #907 ) ;
#11868=DIRECTION ( 'NONE',  ( 1.000000000000000000, 0.000000000000000000, 0.000000000000000000 ) ) ;
#11873=CARTESIAN_POINT ( 'NONE',  ( 0.000000000000000000, 0.000000000000000000, 46.00000000000000711 ) ) ;
#11876=EDGE_CURVE ( 'NONE', #3628, #798, #13774, .T. ) ;
#11878=AXIS2_PLACEMENT_3D ( 'NONE', #3016, #14569, #8193 ) ;
#11882=LINE ( 'NONE', #559, #5767 ) ;
#11884=ORIENTED_EDGE ( 'NONE', *, *, #13216, .F. ) ;
#11892=ORIENTED_EDGE ( 'NONE', *, *, #13222, .F. ) ;
#11959=CARTESIAN_POINT ( 'NONE',  ( 6.249999999999902300, -10.82531754730554496, 169.0000000000000000 ) ) ;
#11963=PRODUCT_DEFINITION_CONTEXT ( 'detailed design', #189, 'design' ) ;
#11968=EDGE_CURVE ( 'NONE', #20902, #4551, #12339, .T. ) ;
#11972=VERTEX_POINT ( 'NONE', #12353 ) ;
#12008=ADVANCED_FACE ( 'NONE', ( #17330 ), #20605, .F. ) ;
#12021=ORIENTED_EDGE ( 'NONE', *, *, #18801, .T. ) ;
#12040=CARTESIAN_POINT ( 'NONE',  ( 7.500000000000000000, 9.184850993605147944E-16, 166.0000000000000000 ) ) ;
#12108=ORIENTED_EDGE ( 'NONE', *, *, #11968, .T. ) ;
#12134=DIRECTION ( 'NONE',  ( -0.000000000000000000, -0.000000000000000000, -1.000000000000000000 ) ) ;
#12136=ORIENTED_EDGE ( 'NONE', *, *, #10229, .F. ) ;
#12191=CARTESIAN_POINT ( 'NONE',  ( 3.599999999999913936, -10.82531754730554496, 166.0000000000000000 ) ) ;
#12216=LINE ( 'NONE', #7438, #1735 ) ;
#12225=AXIS2_PLACEMENT_3D ( 'NONE', #11363, #17839, #14642 ) ;
#12228=EDGE_CURVE ( 'NONE', #12404, #7756, #11644, .T. ) ;
#12259=VERTEX_POINT ( 'NONE', #17754 ) ;
#12287=MECHANICAL_DESIGN_GEOMETRIC_PRESENTATION_REPRESENTATION('',(#18720),#8547);
#12315=DIRECTION ( 'NONE',  ( -1.000000000000000000, 0.000000000000000000, 0.000000000000000000 ) ) ;
#12319=AXIS2_PLACEMENT_3D ( 'NONE', #7358, #15623, #12785 ) ;
#12339=CIRCLE ( 'NONE', #7232, 2.649999999999987477 ) ;
#12342=ORIENTED_EDGE ( 'NONE', *, *, #4404, .F. ) ;
#12353=CARTESIAN_POINT ( 'NONE',  ( 3.600000000000060485, 10.82531754730546147, 169.0000000000000000 ) ) ;
#12355=DIRECTION ( 'NONE',  ( -0.000000000000000000, -0.000000000000000000, 1.000000000000000000 ) ) ;
#12375=ORIENTED_EDGE ( 'NONE', *, *, #6455, .F. ) ;
#12398=EDGE_CURVE ( 'NONE', #798, #7823, #20788, .T. ) ;
#12404=VERTEX_POINT ( 'NONE', #5846 ) ;
#12442=CARTESIAN_POINT ( 'NONE',  ( -12.50000000000000533, 0.000000000000000000, 169.0000000000000000 ) ) ;
#12461=AXIS2_PLACEMENT_3D ( 'NONE', #19474, #3361, #185 ) ;
#12462=CARTESIAN_POINT ( 'NONE',  ( 8.900000000000046541, 10.82531754730546147, 166.0000000000000000 ) ) ;
#12493=DIRECTION ( 'NONE',  ( 1.000000000000000000, 0.000000000000000000, 0.000000000000000000 ) ) ;
#12536=FACE_BOUND ( 'NONE', #14423, .T. ) ;
#12591=AXIS2_PLACEMENT_3D ( 'NONE', #3121, #12884, #1442 ) ;
#12635=CARTESIAN_POINT ( 'NONE',  ( 6.250000000000054179, 10.82531754730546147, 166.0000000000000000 ) ) ;
#12660=DIRECTION ( 'NONE',  ( -0.000000000000000000, -0.000000000000000000, -1.000000000000000000 ) ) ;
#12722=VECTOR ( 'NONE', #10850, 1000.000000000000000 ) ;
#12749=ADVANCED_FACE ( 'NONE', ( #638 ), #17278, .F. ) ;
#12785=DIRECTION ( 'NONE',  ( 1.000000000000000000, 0.000000000000000000, 0.000000000000000000 ) ) ;
#12814=DIRECTION ( 'NONE',  ( -0.000000000000000000, -0.000000000000000000, -1.000000000000000000 ) ) ;
#12840=SHAPE_REPRESENTATION_RELATIONSHIP ( 'NONE' , 'NONE' ,  #7225, #11209 ) ;
#12862=DIRECTION ( 'NONE',  ( 1.000000000000000000, 0.000000000000000000, -0.000000000000000000 ) ) ;
#12884=DIRECTION ( 'NONE',  ( -0.000000000000000000, -0.000000000000000000, -1.000000000000000000 ) ) ;
#12900=CARTESIAN_POINT ( 'NONE',  ( 17.50000000000000355, 0.000000000000000000, 166.0000000000000000 ) ) ;
#12935=VECTOR ( 'NONE', #15870, 1000.000000000000000 ) ;
#12938=( NAMED_UNIT ( * ) SI_UNIT ( $, .STERADIAN. ) SOLID_ANGLE_UNIT ( ) );
#12984=CIRCLE ( 'NONE', #16689, 7.500000000000000000 ) ;
#13001=CARTESIAN_POINT ( 'NONE',  ( 6.249999999999902300, -10.82531754730554496, 166.0000000000000000 ) ) ;
#13012=CARTESIAN_POINT ( 'NONE',  ( -9.850000000000012079, 3.245314017740478073E-16, 166.0000000000000000 ) ) ;
#13043=ADVANCED_FACE ( 'NONE', ( #5575 ), #5161, .F. ) ;
#13087=CIRCLE ( 'NONE', #3922, 2.649999999999992806 ) ;
#13088=VERTEX_POINT ( 'NONE', #396 ) ;
#13098=CARTESIAN_POINT ( 'NONE',  ( 0.000000000000000000, 0.000000000000000000, 166.0000000000000000 ) ) ;
#13106=AXIS2_PLACEMENT_3D ( 'NONE', #709, #6849, #13339 ) ;
#13125=ORIENTED_EDGE ( 'NONE', *, *, #11555, .F. ) ;
#13151=CARTESIAN_POINT ( 'NONE',  ( -17.50000000000000355, 2.143131898507868643E-15, 166.0000000000000000 ) ) ;
#13172=FACE_OUTER_BOUND ( 'NONE', #11838, .T. ) ;
#13182=VERTEX_POINT ( 'NONE', #7714 ) ;
#13215=PRODUCT ( 'output shaft', 'output shaft', '', ( #10036 ) ) ;
#13216=EDGE_CURVE ( 'NONE', #10156, #10605, #10790, .T. ) ;
#13222=EDGE_CURVE ( 'NONE', #13237, #1377, #13087, .T. ) ;
#13237=VERTEX_POINT ( 'NONE', #18948 ) ;
#13303=CIRCLE ( 'NONE', #15955, 2.649999999999987477 ) ;
#13316=DIRECTION ( 'NONE',  ( 0.000000000000000000, 0.000000000000000000, 1.000000000000000000 ) ) ;
#13339=DIRECTION ( 'NONE',  ( -1.000000000000000000, 0.000000000000000000, 0.000000000000000000 ) ) ;
#13429=CIRCLE ( 'NONE', #4281, 2.649999999999993694 ) ;
#13469=CARTESIAN_POINT ( 'NONE',  ( -15.15000000000000036, 3.245314017740477087E-16, 43.00000000000000000 ) ) ;
#13470=VECTOR ( 'NONE', #16098, 1000.000000000000000 ) ;
#13477=ORIENTED_EDGE ( 'NONE', *, *, #10804, .F. ) ;
#13500=EDGE_LOOP ( 'NONE', ( #8125, #6038 ) ) ;
#13504=ADVANCED_FACE ( 'NONE', ( #2261 ), #20370, .F. ) ;
#13511=CIRCLE ( 'NONE', #19255, 2.649999999999987477 ) ;
#13616=VECTOR ( 'NONE', #393, 1000.000000000000000 ) ;
#13632=CIRCLE ( 'NONE', #16009, 17.50000000000000355 ) ;
#13663=AXIS2_PLACEMENT_3D ( 'NONE', #4797, #1643, #17741 ) ;
#13674=CARTESIAN_POINT ( 'NONE',  ( 3.600000000000060485, 10.82531754730546147, 43.00000000000000000 ) ) ;
#13681=AXIS2_PLACEMENT_3D ( 'NONE', #1436, #14369, #6296 ) ;
#13724=CIRCLE ( 'NONE', #11010, 2.649999999999994582 ) ;
#13771=DIRECTION ( 'NONE',  ( -1.000000000000000000, 0.000000000000000000, 0.000000000000000000 ) ) ;
#13774=CIRCLE ( 'NONE', #12319, 17.50000000000000355 ) ;
#13791=ORIENTED_EDGE ( 'NONE', *, *, #33, .F. ) ;
#13874=AXIS2_PLACEMENT_3D ( 'NONE', #16820, #704, #16918 ) ;
#13891=DIRECTION ( 'NONE',  ( -1.000000000000000000, 0.000000000000000000, 0.000000000000000000 ) ) ;
#13894=VERTEX_POINT ( 'NONE', #10291 ) ;
#13985=ORIENTED_EDGE ( 'NONE', *, *, #18633, .F. ) ;
#14012=CIRCLE ( 'NONE', #8576, 17.50000000000000355 ) ;
#14016=ADVANCED_FACE ( 'NONE', ( #15791 ), #10718, .T. ) ;
#14030=CARTESIAN_POINT ( 'NONE',  ( 3.600000000000066702, 10.82531754730546147, 166.0000000000000000 ) ) ;
#14032=PLANE ( 'NONE',  #7808 ) ;
#14037=PLANE ( 'NONE',  #7988 ) ;
#14063=DIRECTION ( 'NONE',  ( 0.000000000000000000, 0.000000000000000000, 1.000000000000000000 ) ) ;
#14067=EDGE_LOOP ( 'NONE', ( #146, #10792 ) ) ;
#14069=CARTESIAN_POINT ( 'NONE',  ( 0.000000000000000000, 0.000000000000000000, 166.0000000000000000 ) ) ;
#14094=ORIENTED_EDGE ( 'NONE', *, *, #14930, .T. ) ;
#14134=ORIENTED_EDGE ( 'NONE', *, *, #49, .F. ) ;
#14138=AXIS2_PLACEMENT_3D ( 'NONE', #16827, #16514, #8760 ) ;
#14141=CARTESIAN_POINT ( 'NONE',  ( 8.899999999999895550, -10.82531754730554496, 169.0000000000000000 ) ) ;
#14144=EDGE_CURVE ( 'NONE', #16612, #7823, #2822, .T. ) ;
#14291=DIRECTION ( 'NONE',  ( -0.000000000000000000, -0.000000000000000000, 1.000000000000000000 ) ) ;
#14297=AXIS2_PLACEMENT_3D ( 'NONE', #5934, #18652, #17388 ) ;
#14306=ADVANCED_FACE ( 'NONE', ( #6630 ), #3151, .T. ) ;
#14321=ORIENTED_EDGE ( 'NONE', *, *, #11876, .T. ) ;
#14325=( NAMED_UNIT ( * ) PLANE_ANGLE_UNIT ( ) SI_UNIT ( $, .RADIAN. ) );
#14327=AXIS2_PLACEMENT_3D ( 'NONE', #5560, #18512, #18613 ) ;
#14347=FACE_BOUND ( 'NONE', #9290, .T. ) ;
#14355=DIRECTION ( 'NONE',  ( -1.000000000000000000, 0.000000000000000000, 0.000000000000000000 ) ) ;
#14369=DIRECTION ( 'NONE',  ( -0.000000000000000000, -0.000000000000000000, -1.000000000000000000 ) ) ;
#14410=EDGE_CURVE ( 'NONE', #6625, #3107, #12984, .T. ) ;
#14423=EDGE_LOOP ( 'NONE', ( #18191, #9738 ) ) ;
#14458=FACE_BOUND ( 'NONE', #13500, .T. ) ;
#14460=AXIS2_PLACEMENT_3D ( 'NONE', #3068, #6140, #13891 ) ;
#14544=DIRECTION ( 'NONE',  ( -0.000000000000000000, -0.000000000000000000, -1.000000000000000000 ) ) ;
#14554=EDGE_CURVE ( 'NONE', #11249, #13182, #6547, .T. ) ;
#14561=ORIENTED_EDGE ( 'NONE', *, *, #20871, .F. ) ;
#14569=DIRECTION ( 'NONE',  ( -0.000000000000000000, -0.000000000000000000, 1.000000000000000000 ) ) ;
#14583=ORIENTED_EDGE ( 'NONE', *, *, #17373, .F. ) ;
#14610=AXIS2_PLACEMENT_3D ( 'NONE', #9446, #15906, #7852 ) ;
#14627=DIRECTION ( 'NONE',  ( -0.000000000000000000, -0.000000000000000000, 1.000000000000000000 ) ) ;
#14636=DIRECTION ( 'NONE',  ( -1.000000000000000000, 0.000000000000000000, 0.000000000000000000 ) ) ;
#14639=EDGE_LOOP ( 'NONE', ( #16094, #11892, #10349, #1725 ) ) ;
#14642=DIRECTION ( 'NONE',  ( 1.000000000000000000, 0.000000000000000000, 0.000000000000000000 ) ) ;
#14807=EDGE_CURVE ( 'NONE', #10156, #8987, #4864, .T. ) ;
#14930=EDGE_CURVE ( 'NONE', #1857, #11867, #5545, .T. ) ;
#14982=ORIENTED_EDGE ( 'NONE', *, *, #4044, .F. ) ;
#15019=VECTOR ( 'NONE', #5015, 1000.000000000000000 ) ;
#15042=CARTESIAN_POINT ( 'NONE',  ( -9.850000000000019185, 3.245314017740474129E-16, 166.0000000000000000 ) ) ;
#15043=DIRECTION ( 'NONE',  ( -0.000000000000000000, -0.000000000000000000, -1.000000000000000000 ) ) ;
#15088=EDGE_CURVE ( 'NONE', #13182, #1857, #10951, .T. ) ;
#15098=AXIS2_PLACEMENT_3D ( 'NONE', #17974, #3442, #4936 ) ;
#15144=CARTESIAN_POINT ( 'NONE',  ( 0.000000000000000000, 0.000000000000000000, 166.0000000000000000 ) ) ;
#15152=AXIS2_PLACEMENT_3D ( 'NONE', #20711, #14063, #10671 ) ;
#15164=CARTESIAN_POINT ( 'NONE',  ( 6.249999999999902300, -10.82531754730554496, 46.00000000000000711 ) ) ;
#15188=CARTESIAN_POINT ( 'NONE',  ( 6.249999999999902300, -10.82531754730554496, 166.0000000000000000 ) ) ;
#15227=FACE_OUTER_BOUND ( 'NONE', #8241, .T. ) ;
#15261=EDGE_LOOP ( 'NONE', ( #118, #10458 ) ) ;
#15285=EDGE_LOOP ( 'NONE', ( #12375, #12136 ) ) ;
#15356=UNCERTAINTY_MEASURE_WITH_UNIT (LENGTH_MEASURE( 1.000000000000000082E-05 ), #3896, 'distance_accuracy_value', 'NONE');
#15364=CIRCLE ( 'NONE', #17404, 2.649999999999993694 ) ;
#15376=ORIENTED_EDGE ( 'NONE', *, *, #17670, .F. ) ;
#15468=EDGE_LOOP ( 'NONE', ( #4182, #4591, #15540, #7261 ) ) ;
#15482=CARTESIAN_POINT ( 'NONE',  ( 8.900000000000041211, 10.82531754730546147, 46.00000000000000711 ) ) ;
#15540=ORIENTED_EDGE ( 'NONE', *, *, #19190, .F. ) ;
#15563=PRODUCT_DEFINITION ( 'UNKNOWN', '', #10323, #11963 ) ;
#15585=ADVANCED_FACE ( 'NONE', ( #15797 ), #7420, .F. ) ;
#15623=DIRECTION ( 'NONE',  ( 0.000000000000000000, 0.000000000000000000, 1.000000000000000000 ) ) ;
#15702=ADVANCED_FACE ( 'NONE', ( #9756 ), #11452, .F. ) ;
#15717=AXIS2_PLACEMENT_3D ( 'NONE', #5863, #2269, #5748 ) ;
#15719=FACE_BOUND ( 'NONE', #17073, .T. ) ;
#15791=FACE_OUTER_BOUND ( 'NONE', #8444, .T. ) ;
#15797=FACE_OUTER_BOUND ( 'NONE', #10460, .T. ) ;
#15870=DIRECTION ( 'NONE',  ( -0.000000000000000000, -0.000000000000000000, 1.000000000000000000 ) ) ;
#15884=EDGE_CURVE ( 'NONE', #5471, #13088, #15364, .T. ) ;
#15899=( LENGTH_UNIT ( ) NAMED_UNIT ( * ) SI_UNIT ( .MILLI., .METRE. ) );
#15906=DIRECTION ( 'NONE',  ( 0.000000000000000000, 0.000000000000000000, -1.000000000000000000 ) ) ;
#15936=FACE_OUTER_BOUND ( 'NONE', #7836, .T. ) ;
#15955=AXIS2_PLACEMENT_3D ( 'NONE', #12635, #9443, #4457 ) ;
#15962=EDGE_CURVE ( 'NONE', #10605, #44, #14012, .T. ) ;
#15965=PLANE ( 'NONE',  #11753 ) ;
#16009=AXIS2_PLACEMENT_3D ( 'NONE', #9278, #12355, #10970 ) ;
#16094=ORIENTED_EDGE ( 'NONE', *, *, #5126, .F. ) ;
#16098=DIRECTION ( 'NONE',  ( -0.000000000000000000, -0.000000000000000000, -1.000000000000000000 ) ) ;
#16118=FILL_AREA_STYLE ('',( #9654 ) ) ;
#16148=CYLINDRICAL_SURFACE ( 'NONE', #13663, 2.649999999999994582 ) ;
#16160=CARTESIAN_POINT ( 'NONE',  ( -12.50000000000000533, 0.000000000000000000, 166.0000000000000000 ) ) ;
#16232=ORIENTED_EDGE ( 'NONE', *, *, #15962, .F. ) ;
#16328=ADVANCED_FACE ( 'NONE', ( #18835 ), #2513, .T. ) ;
#16395=CARTESIAN_POINT ( 'NONE',  ( 3.600000000000066702, 10.82531754730546147, 46.00000000000000711 ) ) ;
#16397=DIRECTION ( 'NONE',  ( -0.000000000000000000, -0.000000000000000000, 1.000000000000000000 ) ) ;
#16417=CARTESIAN_POINT ( 'NONE',  ( -12.50000000000000533, 0.000000000000000000, 46.00000000000000711 ) ) ;
#16490=EDGE_CURVE ( 'NONE', #8932, #10942, #20050, .T. ) ;
#16494=ORIENTED_EDGE ( 'NONE', *, *, #9973, .T. ) ;
#16502=CIRCLE ( 'NONE', #15152, 2.649999999999993694 ) ;
#16511=CARTESIAN_POINT ( 'NONE',  ( 8.899999999999895550, -10.82531754730554496, 46.00000000000000711 ) ) ;
#16514=DIRECTION ( 'NONE',  ( -0.000000000000000000, -0.000000000000000000, 1.000000000000000000 ) ) ;
#16612=VERTEX_POINT ( 'NONE', #8734 ) ;
#16617=AXIS2_PLACEMENT_3D ( 'NONE', #15164, #2128, #11868 ) ;
#16640=CYLINDRICAL_SURFACE ( 'NONE', #16617, 2.649999999999993694 ) ;
#16666=ORIENTED_EDGE ( 'NONE', *, *, #18562, .F. ) ;
#16667=CARTESIAN_POINT ( 'NONE',  ( 8.900000000000046541, 10.82531754730546147, 169.0000000000000000 ) ) ;
#16689=AXIS2_PLACEMENT_3D ( 'NONE', #6183, #4493, #7567 ) ;
#16776=CARTESIAN_POINT ( 'NONE',  ( 3.599999999999913936, -10.82531754730554496, 46.00000000000000711 ) ) ;
#16807=STYLED_ITEM ( 'NONE', ( #7635 ), #11209 ) ;
#16820=CARTESIAN_POINT ( 'NONE',  ( 6.249999999999902300, -10.82531754730554496, 43.00000000000000000 ) ) ;
#16827=CARTESIAN_POINT ( 'NONE',  ( 6.250000000000054179, 10.82531754730546147, 46.00000000000000711 ) ) ;
#16857=ORIENTED_EDGE ( 'NONE', *, *, #4539, .T. ) ;
#16918=DIRECTION ( 'NONE',  ( 1.000000000000000000, 0.000000000000000000, 0.000000000000000000 ) ) ;
#16938=( NAMED_UNIT ( * ) SI_UNIT ( $, .STERADIAN. ) SOLID_ANGLE_UNIT ( ) );
#16963=CIRCLE ( 'NONE', #19668, 2.649999999999988365 ) ;
#16992=EDGE_CURVE ( 'NONE', #9250, #2396, #1391, .T. ) ;
#17044=ORIENTED_EDGE ( 'NONE', *, *, #5799, .F. ) ;
#17073=EDGE_LOOP ( 'NONE', ( #8526, #10773 ) ) ;
#17136=ORIENTED_EDGE ( 'NONE', *, *, #8027, .F. ) ;
#17278=CYLINDRICAL_SURFACE ( 'NONE', #5655, 2.649999999999992806 ) ;
#17330=FACE_OUTER_BOUND ( 'NONE', #18517, .T. ) ;
#17352=DIRECTION ( 'NONE',  ( -0.000000000000000000, -0.000000000000000000, 1.000000000000000000 ) ) ;
#17373=EDGE_CURVE ( 'NONE', #13894, #4175, #19338, .T. ) ;
#17380=EDGE_LOOP ( 'NONE', ( #3576, #3260, #10174, #14982 ) ) ;
#17388=DIRECTION ( 'NONE',  ( 1.000000000000000000, 0.000000000000000000, 0.000000000000000000 ) ) ;
#17404=AXIS2_PLACEMENT_3D ( 'NONE', #11959, #6971, #13771 ) ;
#17421=FACE_OUTER_BOUND ( 'NONE', #10581, .T. ) ;
#17444=ORIENTED_EDGE ( 'NONE', *, *, #1730, .F. ) ;
#17466=CARTESIAN_POINT ( 'NONE',  ( 6.250000000000054179, 10.82531754730546147, 43.00000000000000000 ) ) ;
#17476=CARTESIAN_POINT ( 'NONE',  ( 17.50000000000000355, 2.143131898507868643E-15, 43.00000000000000000 ) ) ;
#17515=DIRECTION ( 'NONE',  ( 1.000000000000000000, 0.000000000000000000, 0.000000000000000000 ) ) ;
#17557=CARTESIAN_POINT ( 'NONE',  ( -9.850000000000019185, 0.000000000000000000, 46.00000000000000711 ) ) ;
#17660=ORIENTED_EDGE ( 'NONE', *, *, #15088, .F. ) ;
#17668=FACE_BOUND ( 'NONE', #6759, .T. ) ;
#17670=EDGE_CURVE ( 'NONE', #12259, #6658, #4034, .T. ) ;
#17712=VECTOR ( 'NONE', #4609, 1000.000000000000000 ) ;
#17741=DIRECTION ( 'NONE',  ( 1.000000000000000000, 0.000000000000000000, 0.000000000000000000 ) ) ;
#17754=CARTESIAN_POINT ( 'NONE',  ( 8.899999999999895550, -10.82531754730554496, 43.00000000000000000 ) ) ;
#17812=ORIENTED_EDGE ( 'NONE', *, *, #12398, .F. ) ;
#17839=DIRECTION ( 'NONE',  ( 0.000000000000000000, 0.000000000000000000, 1.000000000000000000 ) ) ;
#17870=AXIS2_PLACEMENT_3D ( 'NONE', #2545, #1566, #3138 ) ;
#17974=CARTESIAN_POINT ( 'NONE',  ( 0.000000000000000000, 0.000000000000000000, 169.0000000000000000 ) ) ;
#17977=FACE_BOUND ( 'NONE', #15285, .T. ) ;
#17992=CARTESIAN_POINT ( 'NONE',  ( 17.50000000000000355, 0.000000000000000000, 169.0000000000000000 ) ) ;
#18017=CIRCLE ( 'NONE', #8871, 2.649999999999993694 ) ;
#18092=CARTESIAN_POINT ( 'NONE',  ( 7.500000000000000000, 9.184850993605147944E-16, 46.00000000000000711 ) ) ;
#18101=LINE ( 'NONE', #8239, #5490 ) ;
#18107=CARTESIAN_POINT ( 'NONE',  ( -7.500000000000000000, 0.000000000000000000, 46.00000000000000711 ) ) ;
#18151=CARTESIAN_POINT ( 'NONE',  ( 0.000000000000000000, 0.000000000000000000, 166.0000000000000000 ) ) ;
#18173=EDGE_CURVE ( 'NONE', #5471, #8014, #8394, .T. ) ;
#18191=ORIENTED_EDGE ( 'NONE', *, *, #8962, .T. ) ;
#18214=DIRECTION ( 'NONE',  ( 0.000000000000000000, 0.000000000000000000, 1.000000000000000000 ) ) ;
#18249=DIRECTION ( 'NONE',  ( -0.000000000000000000, -0.000000000000000000, -1.000000000000000000 ) ) ;
#18346=CIRCLE ( 'NONE', #12591, 2.649999999999988365 ) ;
#18365=DIRECTION ( 'NONE',  ( -0.000000000000000000, -0.000000000000000000, -1.000000000000000000 ) ) ;
#18386=CARTESIAN_POINT ( 'NONE',  ( -17.50000000000000355, 0.000000000000000000, 46.00000000000000711 ) ) ;
#18412=AXIS2_PLACEMENT_3D ( 'NONE', #16160, #11689, #6705 ) ;
#18428=EDGE_CURVE ( 'NONE', #8932, #6625, #11882, .T. ) ;
#18507=CIRCLE ( 'NONE', #5972, 17.50000000000000355 ) ;
#18512=DIRECTION ( 'NONE',  ( 0.000000000000000000, 0.000000000000000000, -1.000000000000000000 ) ) ;
#18517=EDGE_LOOP ( 'NONE', ( #5219, #10720, #2198, #16494 ) ) ;
#18562=EDGE_CURVE ( 'NONE', #11867, #1857, #13511, .T. ) ;
#18613=DIRECTION ( 'NONE',  ( -1.000000000000000000, 0.000000000000000000, 0.000000000000000000 ) ) ;
#18630=ORIENTED_EDGE ( 'NONE', *, *, #18562, .T. ) ;
#18633=EDGE_CURVE ( 'NONE', #13088, #5471, #13429, .T. ) ;
#18652=DIRECTION ( 'NONE',  ( -0.000000000000000000, -0.000000000000000000, 1.000000000000000000 ) ) ;
#18660=( NAMED_UNIT ( * ) PLANE_ANGLE_UNIT ( ) SI_UNIT ( $, .RADIAN. ) );
#18714=CARTESIAN_POINT ( 'NONE',  ( 8.899999999999890221, -10.82531754730554496, 166.0000000000000000 ) ) ;
#18720=STYLED_ITEM ( 'NONE', ( #416 ), #10194 ) ;
#18774=CARTESIAN_POINT ( 'NONE',  ( 0.000000000000000000, 0.000000000000000000, 43.00000000000000000 ) ) ;
#18790=DIRECTION ( 'NONE',  ( -0.000000000000000000, -0.000000000000000000, -1.000000000000000000 ) ) ;
#18792=EDGE_LOOP ( 'NONE', ( #3769, #10286 ) ) ;
#18801=EDGE_CURVE ( 'NONE', #1377, #13237, #4981, .T. ) ;
#18835=FACE_OUTER_BOUND ( 'NONE', #15468, .T. ) ;
#18853=ORIENTED_EDGE ( 'NONE', *, *, #12228, .F. ) ;
#18864=COLOUR_RGB ( '', 0.40784314, 0.44705882, 0.49803922) ;
#18870=PLANE ( 'NONE',  #17870 ) ;
#18910=DIRECTION ( 'NONE',  ( 0.000000000000000000, 0.000000000000000000, 1.000000000000000000 ) ) ;
#18913=CARTESIAN_POINT ( 'NONE',  ( -9.850000000000012079, 0.000000000000000000, 46.00000000000000711 ) ) ;
#18948=CARTESIAN_POINT ( 'NONE',  ( 8.900000000000046541, 10.82531754730546147, 43.00000000000000000 ) ) ;
#18996=AXIS2_PLACEMENT_3D ( 'NONE', #15188, #994, #20153 ) ;
#19068=ADVANCED_FACE ( 'NONE', ( #17668, #4112, #20448, #10598, #6414 ), #18870, .T. ) ;
#19071=LINE ( 'NONE', #4547, #13470 ) ;
#19083=ORIENTED_EDGE ( 'NONE', *, *, #18801, .F. ) ;
#19114=CARTESIAN_POINT ( 'NONE',  ( 0.000000000000000000, 0.000000000000000000, 169.0000000000000000 ) ) ;
#19127=CARTESIAN_POINT ( 'NONE',  ( 6.250000000000054179, 10.82531754730546147, 166.0000000000000000 ) ) ;
#19190=EDGE_CURVE ( 'NONE', #44, #10605, #6627, .T. ) ;
#19255=AXIS2_PLACEMENT_3D ( 'NONE', #4575, #9132, #17515 ) ;
#19286=EDGE_CURVE ( 'NONE', #5950, #8014, #11380, .T. ) ;
#19299=EDGE_LOOP ( 'NONE', ( #14321, #5091 ) ) ;
#19321=DIRECTION ( 'NONE',  ( 0.000000000000000000, 0.000000000000000000, 1.000000000000000000 ) ) ;
#19328=EDGE_LOOP ( 'NONE', ( #8278, #12342 ) ) ;
#19332=EDGE_CURVE ( 'NONE', #3628, #16612, #20280, .T. ) ;
#19334=VECTOR ( 'NONE', #9014, 1000.000000000000000 ) ;
#19338=CIRCLE ( 'NONE', #14610, 2.649999999999994582 ) ;
#19400=AXIS2_PLACEMENT_3D ( 'NONE', #1302, #1396, #7522 ) ;
#19474=CARTESIAN_POINT ( 'NONE',  ( 0.000000000000000000, 0.000000000000000000, 0.000000000000000000 ) ) ;
#19626=CARTESIAN_POINT ( 'NONE',  ( -12.50000000000000533, 0.000000000000000000, 43.00000000000000000 ) ) ;
#19629=CYLINDRICAL_SURFACE ( 'NONE', #11878, 17.50000000000000355 ) ;
#19668=AXIS2_PLACEMENT_3D ( 'NONE', #5287, #5485, #5699 ) ;
#19800=ORIENTED_EDGE ( 'NONE', *, *, #19830, .F. ) ;
#19806=CIRCLE ( 'NONE', #10690, 2.649999999999987477 ) ;
#19830=EDGE_CURVE ( 'NONE', #798, #3628, #18507, .T. ) ;
#19871=AXIS2_PLACEMENT_3D ( 'NONE', #1046, #14291, #12493 ) ;
#20002=ADVANCED_FACE ( 'NONE', ( #15227 ), #395, .F. ) ;
#20008=AXIS2_PLACEMENT_3D ( 'NONE', #4684, #14544, #14636 ) ;
#20050=CIRCLE ( 'NONE', #10930, 7.500000000000000000 ) ;
#20115=DIRECTION ( 'NONE',  ( -0.000000000000000000, -0.000000000000000000, -1.000000000000000000 ) ) ;
#20126=ORIENTED_EDGE ( 'NONE', *, *, #14554, .F. ) ;
#20153=DIRECTION ( 'NONE',  ( -1.000000000000000000, 0.000000000000000000, 0.000000000000000000 ) ) ;
#20266=EDGE_LOOP ( 'NONE', ( #19800, #6962, #4890, #9906 ) ) ;
#20268=DIRECTION ( 'NONE',  ( -0.000000000000000000, -0.000000000000000000, -1.000000000000000000 ) ) ;
#20280=LINE ( 'NONE', #18386, #208 ) ;
#20304=CARTESIAN_POINT ( 'NONE',  ( -17.50000000000000355, 2.143131898507868643E-15, 166.0000000000000000 ) ) ;
#20326=ADVANCED_FACE ( 'NONE', ( #1868, #3042, #17977, #279, #9614 ), #15965, .T. ) ;
#20355=CARTESIAN_POINT ( 'NONE',  ( 6.250000000000054179, 10.82531754730546147, 46.00000000000000711 ) ) ;
#20370=CYLINDRICAL_SURFACE ( 'NONE', #9411, 2.649999999999993694 ) ;
#20404=VECTOR ( 'NONE', #9595, 1000.000000000000000 ) ;
#20448=FACE_BOUND ( 'NONE', #389, .T. ) ;
#20476=DIRECTION ( 'NONE',  ( -0.000000000000000000, -0.000000000000000000, -1.000000000000000000 ) ) ;
#20521=ORIENTED_EDGE ( 'NONE', *, *, #10894, .F. ) ;
#20531=DIRECTION ( 'NONE',  ( -0.000000000000000000, -0.000000000000000000, 1.000000000000000000 ) ) ;
#20587=CARTESIAN_POINT ( 'NONE',  ( -9.850000000000012079, 3.245314017740477087E-16, 169.0000000000000000 ) ) ;
#20605=CYLINDRICAL_SURFACE ( 'NONE', #13681, 2.649999999999993694 ) ;
#20654=CYLINDRICAL_SURFACE ( 'NONE', #14297, 2.649999999999993694 ) ;
#20659=ORIENTED_EDGE ( 'NONE', *, *, #14807, .T. ) ;
#20687=DIRECTION ( 'NONE',  ( 0.000000000000000000, 0.000000000000000000, -1.000000000000000000 ) ) ;
#20711=CARTESIAN_POINT ( 'NONE',  ( 6.249999999999902300, -10.82531754730554496, 43.00000000000000000 ) ) ;
#20712=LINE ( 'NONE', #3029, #20404 ) ;
#20777=AXIS2_PLACEMENT_3D ( 'NONE', #19626, #19321, #1938 ) ;
#20788=LINE ( 'NONE', #990, #4889 ) ;
#20871=EDGE_CURVE ( 'NONE', #11972, #2396, #19071, .T. ) ;
#20902=VERTEX_POINT ( 'NONE', #16395 ) ;
ENDSEC;
END-ISO-10303-21;
